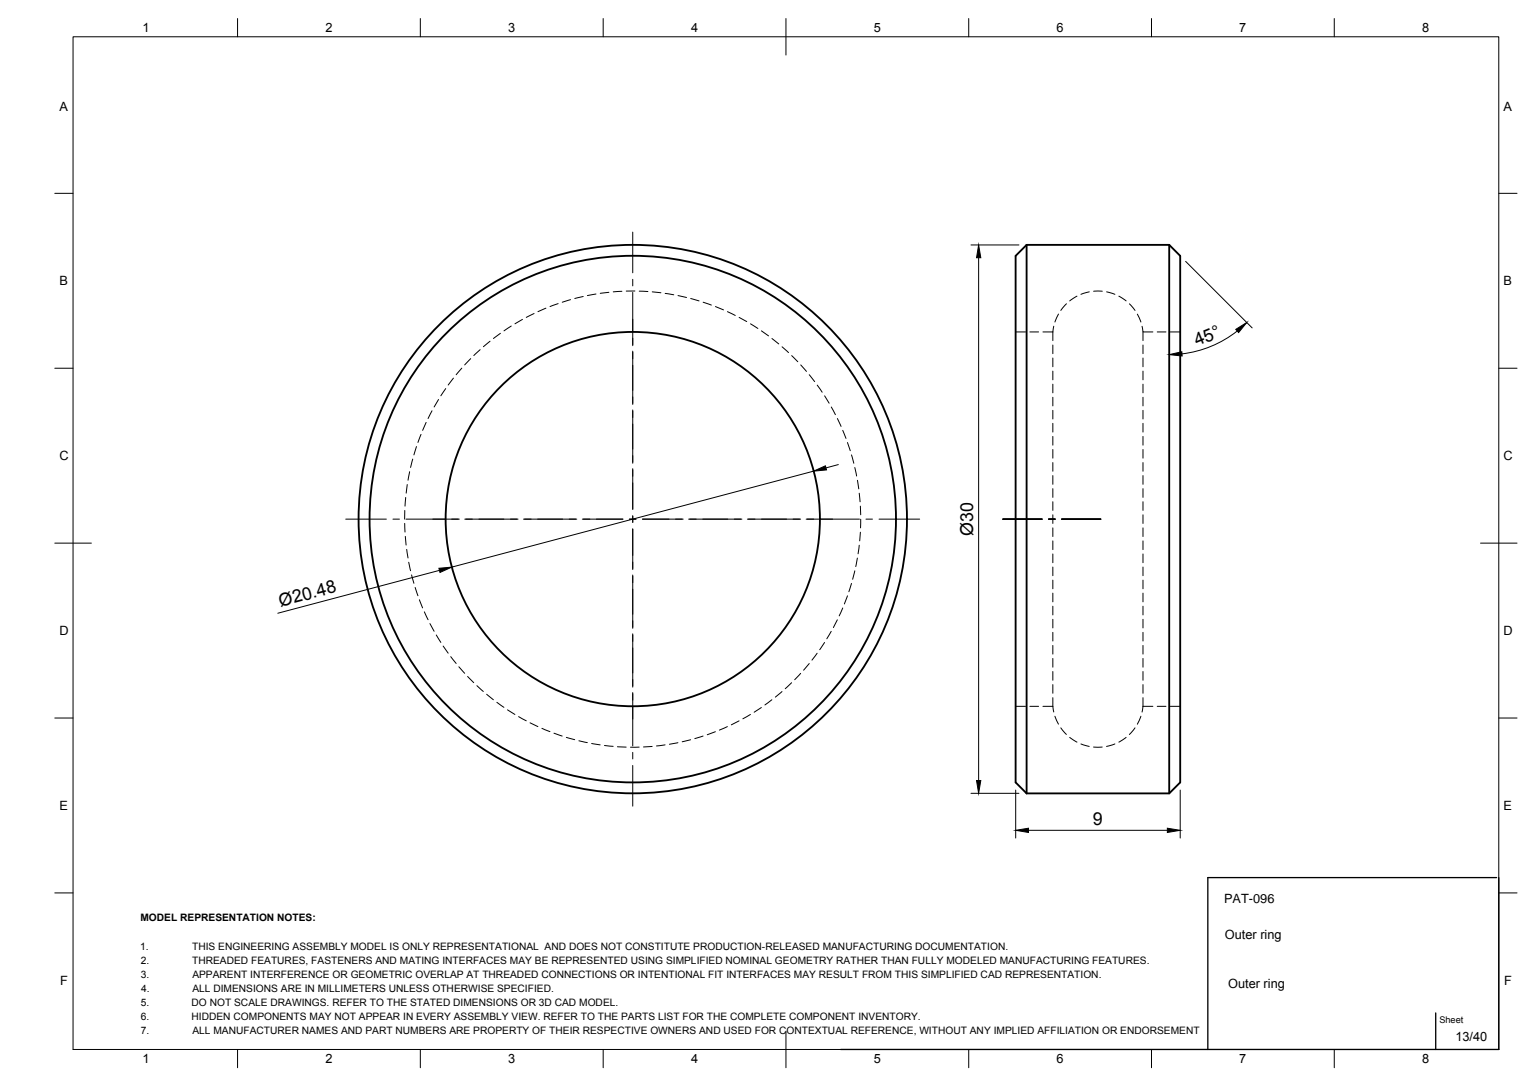
ISO-10303-21;
HEADER;
/* Generated by software containing ST-Developer
 * from STEP Tools, Inc. (www.steptools.com) 
 */

FILE_DESCRIPTION(
/* description */ ('PAT-096'),
/* implementation_level */ '2;1');

FILE_NAME(
/* name */ 'Outer ring.step',
/* time_stamp */ '2026-10-29T17:03:14-07:00',
/* author */ (''),
/* organization */ (''),
/* preprocessor_version */ 'ST-DEVELOPER v20.2',
/* originating_system */ 'Autodesk Translation Framework v15.17.0.0',
/* authorisation */ '');

FILE_SCHEMA (('AUTOMOTIVE_DESIGN { 1 0 10303 214 3 1 1 }'));
ENDSEC;

DATA;
#10=MECHANICAL_DESIGN_GEOMETRIC_PRESENTATION_REPRESENTATION('',(#403),#10650);
#280=TOROIDAL_SURFACE('',#6105,1.,0.247676);
#317=CONICAL_SURFACE('',#6116,1.47,0.785398163397449);
#318=CONICAL_SURFACE('',#6120,1.47,0.785398163397449);
#341=SHAPE_REPRESENTATION_RELATIONSHIP('SRR','None',#10802,#372);
#372=ADVANCED_BREP_SHAPE_REPRESENTATION('',(#441),#10620);
#403=STYLED_ITEM('',(#11064),#441);
#441=MANIFOLD_SOLID_BREP('Body1',#5537);
#525=FACE_BOUND('',#1266,.T.);
#526=FACE_BOUND('',#1271,.T.);
#650=PLANE('',#6113);
#651=PLANE('',#6122);
#875=FACE_OUTER_BOUND('',#1263,.T.);
#876=FACE_OUTER_BOUND('',#1264,.T.);
#877=FACE_OUTER_BOUND('',#1265,.T.);
#878=FACE_OUTER_BOUND('',#1267,.T.);
#879=FACE_OUTER_BOUND('',#1268,.T.);
#880=FACE_OUTER_BOUND('',#1269,.T.);
#881=FACE_OUTER_BOUND('',#1270,.T.);
#882=FACE_OUTER_BOUND('',#1272,.T.);
#1263=EDGE_LOOP('',(#4075,#4076,#4077,#4078,#4079,#4080));
#1264=EDGE_LOOP('',(#4081,#4082,#4083,#4084,#4085));
#1265=EDGE_LOOP('',(#4086));
#1266=EDGE_LOOP('',(#4087));
#1267=EDGE_LOOP('',(#4088,#4089,#4090,#4091));
#1268=EDGE_LOOP('',(#4092,#4093,#4094,#4095));
#1269=EDGE_LOOP('',(#4096,#4097,#4098,#4099));
#1270=EDGE_LOOP('',(#4100));
#1271=EDGE_LOOP('',(#4101));
#1272=EDGE_LOOP('',(#4102,#4103,#4104,#4105,#4106));
#1681=LINE('',#8986,#2010);
#1682=LINE('',#8995,#2011);
#1683=LINE('',#8999,#2012);
#1684=LINE('',#9003,#2013);
#1685=LINE('',#9006,#2014);
#2010=VECTOR('',#7147,1.023815);
#2011=VECTOR('',#7158,1.47);
#2012=VECTOR('',#7163,1.5);
#2013=VECTOR('',#7168,1.47);
#2014=VECTOR('',#7173,1.023815);
#2355=CIRCLE('',#6106,1.023815);
#2356=CIRCLE('',#6107,1.023815);
#2357=CIRCLE('',#6108,0.247676);
#2358=CIRCLE('',#6109,1.023815);
#2359=CIRCLE('',#6110,1.023815);
#2360=CIRCLE('',#6112,1.023815);
#2361=CIRCLE('',#6114,1.44);
#2362=CIRCLE('',#6115,1.023815);
#2363=CIRCLE('',#6117,1.5);
#2364=CIRCLE('',#6119,1.5);
#2365=CIRCLE('',#6121,1.44);
#2697=VERTEX_POINT('',#8974);
#2698=VERTEX_POINT('',#8975);
#2699=VERTEX_POINT('',#8978);
#2700=VERTEX_POINT('',#8980);
#2701=VERTEX_POINT('',#8984);
#2702=VERTEX_POINT('',#8988);
#2703=VERTEX_POINT('',#8990);
#2704=VERTEX_POINT('',#8993);
#2705=VERTEX_POINT('',#8997);
#2706=VERTEX_POINT('',#9001);
#3216=EDGE_CURVE('',#2697,#2698,#2355,.T.);
#3217=EDGE_CURVE('',#2698,#2697,#2356,.T.);
#3218=EDGE_CURVE('',#2698,#2699,#2357,.T.);
#3219=EDGE_CURVE('',#2700,#2699,#2358,.T.);
#3220=EDGE_CURVE('',#2699,#2700,#2359,.T.);
#3221=EDGE_CURVE('',#2701,#2701,#2360,.T.);
#3222=EDGE_CURVE('',#2701,#2700,#1681,.T.);
#3223=EDGE_CURVE('',#2702,#2702,#2361,.T.);
#3224=EDGE_CURVE('',#2703,#2703,#2362,.T.);
#3225=EDGE_CURVE('',#2704,#2704,#2363,.T.);
#3226=EDGE_CURVE('',#2704,#2702,#1682,.T.);
#3227=EDGE_CURVE('',#2705,#2705,#2364,.T.);
#3228=EDGE_CURVE('',#2705,#2704,#1683,.T.);
#3229=EDGE_CURVE('',#2706,#2706,#2365,.T.);
#3230=EDGE_CURVE('',#2706,#2705,#1684,.T.);
#3231=EDGE_CURVE('',#2697,#2703,#1685,.T.);
#4075=ORIENTED_EDGE('',*,*,#3216,.F.);
#4076=ORIENTED_EDGE('',*,*,#3217,.F.);
#4077=ORIENTED_EDGE('',*,*,#3218,.T.);
#4078=ORIENTED_EDGE('',*,*,#3219,.F.);
#4079=ORIENTED_EDGE('',*,*,#3220,.F.);
#4080=ORIENTED_EDGE('',*,*,#3218,.F.);
#4081=ORIENTED_EDGE('',*,*,#3221,.T.);
#4082=ORIENTED_EDGE('',*,*,#3222,.T.);
#4083=ORIENTED_EDGE('',*,*,#3219,.T.);
#4084=ORIENTED_EDGE('',*,*,#3220,.T.);
#4085=ORIENTED_EDGE('',*,*,#3222,.F.);
#4086=ORIENTED_EDGE('',*,*,#3223,.F.);
#4087=ORIENTED_EDGE('',*,*,#3224,.T.);
#4088=ORIENTED_EDGE('',*,*,#3225,.F.);
#4089=ORIENTED_EDGE('',*,*,#3226,.T.);
#4090=ORIENTED_EDGE('',*,*,#3223,.T.);
#4091=ORIENTED_EDGE('',*,*,#3226,.F.);
#4092=ORIENTED_EDGE('',*,*,#3227,.F.);
#4093=ORIENTED_EDGE('',*,*,#3228,.T.);
#4094=ORIENTED_EDGE('',*,*,#3225,.T.);
#4095=ORIENTED_EDGE('',*,*,#3228,.F.);
#4096=ORIENTED_EDGE('',*,*,#3229,.F.);
#4097=ORIENTED_EDGE('',*,*,#3230,.T.);
#4098=ORIENTED_EDGE('',*,*,#3227,.T.);
#4099=ORIENTED_EDGE('',*,*,#3230,.F.);
#4100=ORIENTED_EDGE('',*,*,#3229,.T.);
#4101=ORIENTED_EDGE('',*,*,#3221,.F.);
#4102=ORIENTED_EDGE('',*,*,#3216,.T.);
#4103=ORIENTED_EDGE('',*,*,#3217,.T.);
#4104=ORIENTED_EDGE('',*,*,#3231,.T.);
#4105=ORIENTED_EDGE('',*,*,#3224,.F.);
#4106=ORIENTED_EDGE('',*,*,#3231,.F.);
#5114=CYLINDRICAL_SURFACE('',#6111,1.023815);
#5115=CYLINDRICAL_SURFACE('',#6118,1.5);
#5116=CYLINDRICAL_SURFACE('',#6123,1.023815);
#5280=ADVANCED_FACE('',(#875),#280,.F.);
#5281=ADVANCED_FACE('',(#876),#5114,.F.);
#5282=ADVANCED_FACE('',(#877,#525),#650,.T.);
#5283=ADVANCED_FACE('',(#878),#317,.T.);
#5284=ADVANCED_FACE('',(#879),#5115,.T.);
#5285=ADVANCED_FACE('',(#880),#318,.T.);
#5286=ADVANCED_FACE('',(#881,#526),#651,.T.);
#5287=ADVANCED_FACE('',(#882),#5116,.F.);
#5537=CLOSED_SHELL('',(#5280,#5281,#5282,#5283,#5284,#5285,#5286,#5287));
#6104=AXIS2_PLACEMENT_3D('',#8972,#7129,#7130);
#6105=AXIS2_PLACEMENT_3D('',#8973,#7131,#7132);
#6106=AXIS2_PLACEMENT_3D('',#8976,#7133,#7134);
#6107=AXIS2_PLACEMENT_3D('',#8977,#7135,#7136);
#6108=AXIS2_PLACEMENT_3D('',#8979,#7137,#7138);
#6109=AXIS2_PLACEMENT_3D('',#8981,#7139,#7140);
#6110=AXIS2_PLACEMENT_3D('',#8982,#7141,#7142);
#6111=AXIS2_PLACEMENT_3D('',#8983,#7143,#7144);
#6112=AXIS2_PLACEMENT_3D('',#8985,#7145,#7146);
#6113=AXIS2_PLACEMENT_3D('',#8987,#7148,#7149);
#6114=AXIS2_PLACEMENT_3D('',#8989,#7150,#7151);
#6115=AXIS2_PLACEMENT_3D('',#8991,#7152,#7153);
#6116=AXIS2_PLACEMENT_3D('',#8992,#7154,#7155);
#6117=AXIS2_PLACEMENT_3D('',#8994,#7156,#7157);
#6118=AXIS2_PLACEMENT_3D('',#8996,#7159,#7160);
#6119=AXIS2_PLACEMENT_3D('',#8998,#7161,#7162);
#6120=AXIS2_PLACEMENT_3D('',#9000,#7164,#7165);
#6121=AXIS2_PLACEMENT_3D('',#9002,#7166,#7167);
#6122=AXIS2_PLACEMENT_3D('',#9004,#7169,#7170);
#6123=AXIS2_PLACEMENT_3D('',#9005,#7171,#7172);
#7129=DIRECTION('axis',(0.,0.,1.));
#7130=DIRECTION('refdir',(1.,0.,0.));
#7131=DIRECTION('center_axis',(0.,-1.,0.));
#7132=DIRECTION('ref_axis',(0.,0.,-1.));
#7133=DIRECTION('center_axis',(0.,-1.,0.));
#7134=DIRECTION('ref_axis',(1.,0.,0.));
#7135=DIRECTION('center_axis',(0.,-1.,0.));
#7136=DIRECTION('ref_axis',(1.,0.,0.));
#7137=DIRECTION('center_axis',(1.,0.,1.22464679914735E-16));
#7138=DIRECTION('ref_axis',(-1.22464679914735E-16,0.,1.));
#7139=DIRECTION('center_axis',(0.,1.,0.));
#7140=DIRECTION('ref_axis',(1.,0.,0.));
#7141=DIRECTION('center_axis',(0.,1.,0.));
#7142=DIRECTION('ref_axis',(1.,0.,0.));
#7143=DIRECTION('center_axis',(0.,-1.,0.));
#7144=DIRECTION('ref_axis',(1.,0.,0.));
#7145=DIRECTION('center_axis',(0.,-1.,0.));
#7146=DIRECTION('ref_axis',(1.,0.,0.));
#7147=DIRECTION('',(0.,1.,0.));
#7148=DIRECTION('center_axis',(0.,1.,0.));
#7149=DIRECTION('ref_axis',(0.,0.,1.));
#7150=DIRECTION('center_axis',(0.,-1.,0.));
#7151=DIRECTION('ref_axis',(1.,0.,0.));
#7152=DIRECTION('center_axis',(0.,-1.,0.));
#7153=DIRECTION('ref_axis',(1.,0.,0.));
#7154=DIRECTION('center_axis',(0.,-1.,0.));
#7155=DIRECTION('ref_axis',(1.,0.,0.));
#7156=DIRECTION('center_axis',(0.,-1.,0.));
#7157=DIRECTION('ref_axis',(1.,0.,0.));
#7158=DIRECTION('',(0.707106781186548,0.707106781186547,8.65956056235494E-17));
#7159=DIRECTION('center_axis',(0.,-1.,0.));
#7160=DIRECTION('ref_axis',(1.,0.,0.));
#7161=DIRECTION('center_axis',(0.,-1.,0.));
#7162=DIRECTION('ref_axis',(1.,0.,0.));
#7163=DIRECTION('',(0.,1.,0.));
#7164=DIRECTION('center_axis',(0.,1.,0.));
#7165=DIRECTION('ref_axis',(1.,0.,0.));
#7166=DIRECTION('center_axis',(0.,-1.,0.));
#7167=DIRECTION('ref_axis',(1.,0.,0.));
#7168=DIRECTION('',(-0.707106781186548,0.707106781186547,-8.65956056235494E-17));
#7169=DIRECTION('center_axis',(0.,-1.,0.));
#7170=DIRECTION('ref_axis',(0.,0.,-1.));
#7171=DIRECTION('center_axis',(0.,-1.,0.));
#7172=DIRECTION('ref_axis',(1.,0.,0.));
#7173=DIRECTION('',(0.,1.,0.));
#8972=CARTESIAN_POINT('',(0.,0.,0.));
#8973=CARTESIAN_POINT('Origin',(0.,0.,0.));
#8974=CARTESIAN_POINT('',(-1.023815,0.246528389340863,-1.25381176266905E-16));
#8975=CARTESIAN_POINT('',(-1.25381176266905E-16,0.246528389340863,1.023815));
#8976=CARTESIAN_POINT('Origin',(0.,0.246528389340863,0.));
#8977=CARTESIAN_POINT('Origin',(0.,0.246528389340863,0.));
#8978=CARTESIAN_POINT('',(-1.25381176266905E-16,-0.246528389340863,1.023815));
#8979=CARTESIAN_POINT('Origin',(-1.22464679914735E-16,0.,1.));
#8980=CARTESIAN_POINT('',(-1.023815,-0.246528389340863,1.25381176266905E-16));
#8981=CARTESIAN_POINT('Origin',(0.,-0.246528389340863,0.));
#8982=CARTESIAN_POINT('Origin',(0.,-0.246528389340863,0.));
#8983=CARTESIAN_POINT('Origin',(0.,0.,0.));
#8984=CARTESIAN_POINT('',(-1.023815,-0.45,-1.25381176266905E-16));
#8985=CARTESIAN_POINT('Origin',(0.,-0.45,0.));
#8986=CARTESIAN_POINT('',(-1.023815,0.,-1.25381176266905E-16));
#8987=CARTESIAN_POINT('Origin',(1.44,0.45,0.));
#8988=CARTESIAN_POINT('',(-1.44,0.45,-1.76349139077219E-16));
#8989=CARTESIAN_POINT('Origin',(0.,0.45,0.));
#8990=CARTESIAN_POINT('',(-1.023815,0.45,-1.25381176266905E-16));
#8991=CARTESIAN_POINT('Origin',(0.,0.45,0.));
#8992=CARTESIAN_POINT('Origin',(0.,0.42,0.));
#8993=CARTESIAN_POINT('',(-1.5,0.39,-1.83697019872103E-16));
#8994=CARTESIAN_POINT('Origin',(0.,0.39,0.));
#8995=CARTESIAN_POINT('',(-1.47,0.42,-1.80023079474661E-16));
#8996=CARTESIAN_POINT('Origin',(0.,0.,0.));
#8997=CARTESIAN_POINT('',(-1.5,-0.39,-1.83697019872103E-16));
#8998=CARTESIAN_POINT('Origin',(0.,-0.39,0.));
#8999=CARTESIAN_POINT('',(-1.5,0.,-1.83697019872103E-16));
#9000=CARTESIAN_POINT('Origin',(0.,-0.42,0.));
#9001=CARTESIAN_POINT('',(-1.44,-0.45,-1.76349139077219E-16));
#9002=CARTESIAN_POINT('Origin',(0.,-0.45,0.));
#9003=CARTESIAN_POINT('',(-1.47,-0.42,-1.80023079474661E-16));
#9004=CARTESIAN_POINT('Origin',(1.023815,-0.45,0.));
#9005=CARTESIAN_POINT('Origin',(0.,0.,0.));
#9006=CARTESIAN_POINT('',(-1.023815,0.,-1.25381176266905E-16));
#10581=UNCERTAINTY_MEASURE_WITH_UNIT(LENGTH_MEASURE(0.001),#10651,
'DISTANCE_ACCURACY_VALUE',
'Maximum model space distance between geometric entities at asserted c
onnectivities');
#10611=UNCERTAINTY_MEASURE_WITH_UNIT(LENGTH_MEASURE(0.001),#10651,
'DISTANCE_ACCURACY_VALUE',
'Maximum model space distance between geometric entities at asserted c
onnectivities');
#10620=(
GEOMETRIC_REPRESENTATION_CONTEXT(3)
GLOBAL_UNCERTAINTY_ASSIGNED_CONTEXT((#10581))
GLOBAL_UNIT_ASSIGNED_CONTEXT((#10651,#10653,#10654))
REPRESENTATION_CONTEXT('','3D')
);
#10650=(
GEOMETRIC_REPRESENTATION_CONTEXT(3)
GLOBAL_UNCERTAINTY_ASSIGNED_CONTEXT((#10611))
GLOBAL_UNIT_ASSIGNED_CONTEXT((#10651,#10653,#10654))
REPRESENTATION_CONTEXT('','3D')
);
#10651=(
LENGTH_UNIT()
NAMED_UNIT(*)
SI_UNIT(.CENTI.,.METRE.)
);
#10653=(
NAMED_UNIT(*)
PLANE_ANGLE_UNIT()
SI_UNIT($,.RADIAN.)
);
#10654=(
NAMED_UNIT(*)
SI_UNIT($,.STERADIAN.)
SOLID_ANGLE_UNIT()
);
#10663=SHAPE_DEFINITION_REPRESENTATION(#10701,#10802);
#10701=PRODUCT_DEFINITION_SHAPE('',$,#10841);
#10802=SHAPE_REPRESENTATION('',(#6104),#10620);
#10832=PRODUCT_DEFINITION_CONTEXT('part definition',#10948,'design');
#10841=PRODUCT_DEFINITION('Outer ring','Outer ring',#10879,#10832);
#10879=PRODUCT_DEFINITION_FORMATION('',$,#10958);
#10948=APPLICATION_CONTEXT(
'Core Data for Automotive Mechanical Design Process');
#10949=PRODUCT_CONTEXT('part definition',#10948,'mechanical');
#10958=PRODUCT('Outer ring','Outer ring','Outer ring',(#10949));
#11058=COLOUR_RGB('Grey',0.48,0.52,0.57);
#11059=FILL_AREA_STYLE_COLOUR('',#11058);
#11060=FILL_AREA_STYLE('',(#11059));
#11061=SURFACE_STYLE_FILL_AREA(#11060);
#11062=SURFACE_SIDE_STYLE('',(#11061));
#11063=SURFACE_STYLE_USAGE(.BOTH.,#11062);
#11064=PRESENTATION_STYLE_ASSIGNMENT((#11063));
ENDSEC;
END-ISO-10303-21;
